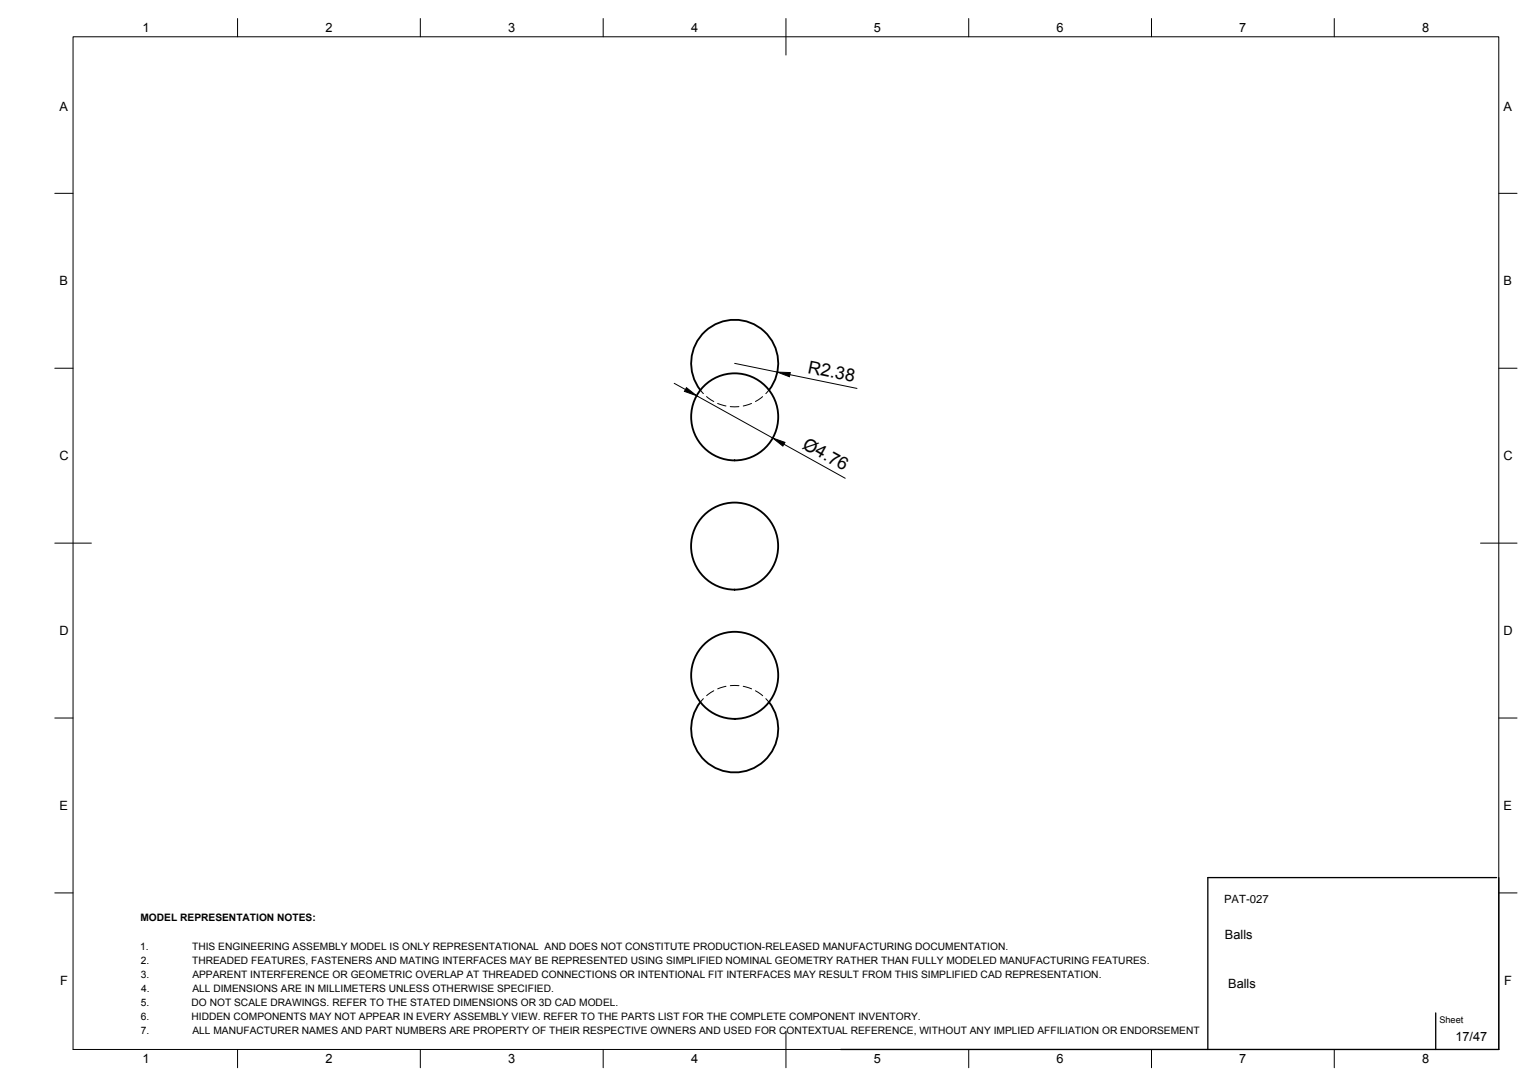
ISO-10303-21;
HEADER;
/* Generated by software containing ST-Developer
 * from STEP Tools, Inc. (www.steptools.com) 
 */

FILE_DESCRIPTION(
/* description */ ('Crank-driven oscillating fan base (mechanism only)'),

/* implementation_level */ '2;1');

FILE_NAME(
/* name */ 'Balls.step',
/* time_stamp */ '2026-10-28T03:25:00-07:00',
/* author */ (''),
/* organization */ (''),
/* preprocessor_version */ 'ST-DEVELOPER v20.2',
/* originating_system */ 'Autodesk Translation Framework v15.17.0.0',
/* authorisation */ '');

FILE_SCHEMA (('AUTOMOTIVE_DESIGN { 1 0 10303 214 3 1 1 }'));
ENDSEC;

DATA;
#10=MECHANICAL_DESIGN_GEOMETRIC_PRESENTATION_REPRESENTATION('',(#448,#449,#450,#451,#452,#453,#454,#455),#11916);
#275=SPHERICAL_SURFACE('',#6871,0.23815);
#276=SPHERICAL_SURFACE('',#6873,0.23815);
#277=SPHERICAL_SURFACE('',#6875,0.23815);
#278=SPHERICAL_SURFACE('',#6877,0.23815);
#279=SPHERICAL_SURFACE('',#6879,0.23815);
#280=SPHERICAL_SURFACE('',#6881,0.23815);
#281=SPHERICAL_SURFACE('',#6883,0.23815);
#282=SPHERICAL_SURFACE('',#6885,0.23815);
#368=SHAPE_REPRESENTATION_RELATIONSHIP('SRR','None',#12093,#408);
#408=ADVANCED_BREP_SHAPE_REPRESENTATION('',(#495,#496,#497,#498,#499,#500,
#501,#502),#11884);
#448=STYLED_ITEM('',(#12375),#495);
#449=STYLED_ITEM('',(#12375),#496);
#450=STYLED_ITEM('',(#12375),#497);
#451=STYLED_ITEM('',(#12375),#498);
#452=STYLED_ITEM('',(#12375),#499);
#453=STYLED_ITEM('',(#12375),#500);
#454=STYLED_ITEM('',(#12375),#501);
#455=STYLED_ITEM('',(#12375),#502);
#495=MANIFOLD_SOLID_BREP('Body1',#6079);
#496=MANIFOLD_SOLID_BREP('Body2',#6080);
#497=MANIFOLD_SOLID_BREP('Body3',#6081);
#498=MANIFOLD_SOLID_BREP('Body4',#6082);
#499=MANIFOLD_SOLID_BREP('Body5',#6083);
#500=MANIFOLD_SOLID_BREP('Body6',#6084);
#501=MANIFOLD_SOLID_BREP('Body7',#6085);
#502=MANIFOLD_SOLID_BREP('Body8',#6086);
#1026=FACE_OUTER_BOUND('',#1482,.T.);
#1027=FACE_OUTER_BOUND('',#1483,.T.);
#1028=FACE_OUTER_BOUND('',#1484,.T.);
#1029=FACE_OUTER_BOUND('',#1485,.T.);
#1030=FACE_OUTER_BOUND('',#1486,.T.);
#1031=FACE_OUTER_BOUND('',#1487,.T.);
#1032=FACE_OUTER_BOUND('',#1488,.T.);
#1033=FACE_OUTER_BOUND('',#1489,.T.);
#1482=EDGE_LOOP('',(#4668,#4669));
#1483=EDGE_LOOP('',(#4670,#4671));
#1484=EDGE_LOOP('',(#4672,#4673));
#1485=EDGE_LOOP('',(#4674,#4675));
#1486=EDGE_LOOP('',(#4676,#4677));
#1487=EDGE_LOOP('',(#4678,#4679));
#1488=EDGE_LOOP('',(#4680,#4681));
#1489=EDGE_LOOP('',(#4682,#4683));
#2621=CIRCLE('',#6872,0.23815);
#2622=CIRCLE('',#6874,0.23815);
#2623=CIRCLE('',#6876,0.23815);
#2624=CIRCLE('',#6878,0.23815);
#2625=CIRCLE('',#6880,0.23815);
#2626=CIRCLE('',#6882,0.23815);
#2627=CIRCLE('',#6884,0.23815);
#2628=CIRCLE('',#6886,0.23815);
#3028=VERTEX_POINT('',#10239);
#3029=VERTEX_POINT('',#10240);
#3030=VERTEX_POINT('',#10243);
#3031=VERTEX_POINT('',#10244);
#3032=VERTEX_POINT('',#10247);
#3033=VERTEX_POINT('',#10248);
#3034=VERTEX_POINT('',#10251);
#3035=VERTEX_POINT('',#10252);
#3036=VERTEX_POINT('',#10255);
#3037=VERTEX_POINT('',#10256);
#3038=VERTEX_POINT('',#10259);
#3039=VERTEX_POINT('',#10260);
#3040=VERTEX_POINT('',#10263);
#3041=VERTEX_POINT('',#10264);
#3042=VERTEX_POINT('',#10267);
#3043=VERTEX_POINT('',#10268);
#3629=EDGE_CURVE('',#3028,#3029,#2621,.T.);
#3630=EDGE_CURVE('',#3030,#3031,#2622,.T.);
#3631=EDGE_CURVE('',#3032,#3033,#2623,.T.);
#3632=EDGE_CURVE('',#3034,#3035,#2624,.T.);
#3633=EDGE_CURVE('',#3036,#3037,#2625,.T.);
#3634=EDGE_CURVE('',#3038,#3039,#2626,.T.);
#3635=EDGE_CURVE('',#3040,#3041,#2627,.T.);
#3636=EDGE_CURVE('',#3042,#3043,#2628,.T.);
#4668=ORIENTED_EDGE('',*,*,#3629,.T.);
#4669=ORIENTED_EDGE('',*,*,#3629,.F.);
#4670=ORIENTED_EDGE('',*,*,#3630,.T.);
#4671=ORIENTED_EDGE('',*,*,#3630,.F.);
#4672=ORIENTED_EDGE('',*,*,#3631,.T.);
#4673=ORIENTED_EDGE('',*,*,#3631,.F.);
#4674=ORIENTED_EDGE('',*,*,#3632,.T.);
#4675=ORIENTED_EDGE('',*,*,#3632,.F.);
#4676=ORIENTED_EDGE('',*,*,#3633,.T.);
#4677=ORIENTED_EDGE('',*,*,#3633,.F.);
#4678=ORIENTED_EDGE('',*,*,#3634,.T.);
#4679=ORIENTED_EDGE('',*,*,#3634,.F.);
#4680=ORIENTED_EDGE('',*,*,#3635,.T.);
#4681=ORIENTED_EDGE('',*,*,#3635,.F.);
#4682=ORIENTED_EDGE('',*,*,#3636,.T.);
#4683=ORIENTED_EDGE('',*,*,#3636,.F.);
#5832=ADVANCED_FACE('',(#1026),#275,.T.);
#5833=ADVANCED_FACE('',(#1027),#276,.T.);
#5834=ADVANCED_FACE('',(#1028),#277,.T.);
#5835=ADVANCED_FACE('',(#1029),#278,.T.);
#5836=ADVANCED_FACE('',(#1030),#279,.T.);
#5837=ADVANCED_FACE('',(#1031),#280,.T.);
#5838=ADVANCED_FACE('',(#1032),#281,.T.);
#5839=ADVANCED_FACE('',(#1033),#282,.T.);
#6079=CLOSED_SHELL('',(#5832));
#6080=CLOSED_SHELL('',(#5833));
#6081=CLOSED_SHELL('',(#5834));
#6082=CLOSED_SHELL('',(#5835));
#6083=CLOSED_SHELL('',(#5836));
#6084=CLOSED_SHELL('',(#5837));
#6085=CLOSED_SHELL('',(#5838));
#6086=CLOSED_SHELL('',(#5839));
#6870=AXIS2_PLACEMENT_3D('',#10237,#8168,#8169);
#6871=AXIS2_PLACEMENT_3D('',#10238,#8170,#8171);
#6872=AXIS2_PLACEMENT_3D('',#10241,#8172,#8173);
#6873=AXIS2_PLACEMENT_3D('',#10242,#8174,#8175);
#6874=AXIS2_PLACEMENT_3D('',#10245,#8176,#8177);
#6875=AXIS2_PLACEMENT_3D('',#10246,#8178,#8179);
#6876=AXIS2_PLACEMENT_3D('',#10249,#8180,#8181);
#6877=AXIS2_PLACEMENT_3D('',#10250,#8182,#8183);
#6878=AXIS2_PLACEMENT_3D('',#10253,#8184,#8185);
#6879=AXIS2_PLACEMENT_3D('',#10254,#8186,#8187);
#6880=AXIS2_PLACEMENT_3D('',#10257,#8188,#8189);
#6881=AXIS2_PLACEMENT_3D('',#10258,#8190,#8191);
#6882=AXIS2_PLACEMENT_3D('',#10261,#8192,#8193);
#6883=AXIS2_PLACEMENT_3D('',#10262,#8194,#8195);
#6884=AXIS2_PLACEMENT_3D('',#10265,#8196,#8197);
#6885=AXIS2_PLACEMENT_3D('',#10266,#8198,#8199);
#6886=AXIS2_PLACEMENT_3D('',#10269,#8200,#8201);
#8168=DIRECTION('axis',(0.,0.,1.));
#8169=DIRECTION('refdir',(1.,0.,0.));
#8170=DIRECTION('center_axis',(0.,0.,1.));
#8171=DIRECTION('ref_axis',(1.,0.,0.));
#8172=DIRECTION('center_axis',(1.22464679914735E-16,-1.,0.));
#8173=DIRECTION('ref_axis',(-1.,-1.22464679914735E-16,0.));
#8174=DIRECTION('center_axis',(0.707106781186548,0.,0.707106781186548));
#8175=DIRECTION('ref_axis',(0.707106781186548,0.,-0.707106781186548));
#8176=DIRECTION('center_axis',(8.65956056235494E-17,-1.,-8.65956056235493E-17));
#8177=DIRECTION('ref_axis',(-0.707106781186547,-1.22464679914735E-16,0.707106781186547));
#8178=DIRECTION('center_axis',(1.,0.,0.));
#8179=DIRECTION('ref_axis',(6.12323399573676E-17,0.,-1.));
#8180=DIRECTION('center_axis',(7.49879891330929E-33,-1.,-1.22464679914735E-16));
#8181=DIRECTION('ref_axis',(-6.12323399573676E-17,-1.22464679914735E-16,
1.));
#8182=DIRECTION('center_axis',(0.707106781186548,0.,-0.707106781186548));
#8183=DIRECTION('ref_axis',(-0.707106781186548,0.,-0.707106781186548));
#8184=DIRECTION('center_axis',(-8.65956056235493E-17,-1.,-8.65956056235494E-17));
#8185=DIRECTION('ref_axis',(0.707106781186547,-1.22464679914735E-16,0.707106781186547));
#8186=DIRECTION('center_axis',(0.,0.,-1.));
#8187=DIRECTION('ref_axis',(-1.,0.,-1.22464679914735E-16));
#8188=DIRECTION('center_axis',(-1.22464679914735E-16,-1.,-1.49975978266186E-32));
#8189=DIRECTION('ref_axis',(1.,-1.22464679914735E-16,1.22464679914735E-16));
#8190=DIRECTION('center_axis',(-0.707106781186547,0.,-0.707106781186548));
#8191=DIRECTION('ref_axis',(-0.707106781186548,0.,0.707106781186547));
#8192=DIRECTION('center_axis',(-8.65956056235493E-17,-1.,8.65956056235493E-17));
#8193=DIRECTION('ref_axis',(0.707106781186548,-1.22464679914735E-16,-0.707106781186547));
#8194=DIRECTION('center_axis',(-1.,0.,0.));
#8195=DIRECTION('ref_axis',(-1.83697019872103E-16,0.,1.));
#8196=DIRECTION('center_axis',(-2.24963967399279E-32,-1.,1.22464679914735E-16));
#8197=DIRECTION('ref_axis',(1.83697019872103E-16,-1.22464679914735E-16,
-1.));
#8198=DIRECTION('center_axis',(-0.707106781186548,0.,0.707106781186548));
#8199=DIRECTION('ref_axis',(0.707106781186547,0.,0.707106781186548));
#8200=DIRECTION('center_axis',(8.65956056235493E-17,-1.,8.65956056235493E-17));
#8201=DIRECTION('ref_axis',(-0.707106781186547,-1.22464679914735E-16,-0.707106781186548));
#10237=CARTESIAN_POINT('',(0.,0.,0.));
#10238=CARTESIAN_POINT('Origin',(1.,0.,0.));
#10239=CARTESIAN_POINT('',(1.,-1.78583896120461E-33,0.23815));
#10240=CARTESIAN_POINT('',(1.,-1.78583896120461E-33,-0.23815));
#10241=CARTESIAN_POINT('Origin',(1.,0.,0.));
#10242=CARTESIAN_POINT('Origin',(0.707106781186548,0.,-0.707106781186547));
#10243=CARTESIAN_POINT('',(0.875504261126124,-1.78583896120461E-33,-0.538709301246971));
#10244=CARTESIAN_POINT('',(0.538709301246971,-1.78583896120461E-33,-0.875504261126124));
#10245=CARTESIAN_POINT('Origin',(0.707106781186548,0.,-0.707106781186547));
#10246=CARTESIAN_POINT('Origin',(6.12323399573677E-17,0.,-1.));
#10247=CARTESIAN_POINT('',(0.23815,-1.78583896120461E-33,-1.));
#10248=CARTESIAN_POINT('',(-0.23815,-1.78583896120461E-33,-1.));
#10249=CARTESIAN_POINT('Origin',(6.12323399573677E-17,0.,-1.));
#10250=CARTESIAN_POINT('Origin',(-0.707106781186547,0.,-0.707106781186548));
#10251=CARTESIAN_POINT('',(-0.538709301246971,-1.78583896120461E-33,-0.875504261126124));
#10252=CARTESIAN_POINT('',(-0.875504261126124,-1.78583896120461E-33,-0.538709301246971));
#10253=CARTESIAN_POINT('Origin',(-0.707106781186547,0.,-0.707106781186548));
#10254=CARTESIAN_POINT('Origin',(-1.,0.,-1.22464679914735E-16));
#10255=CARTESIAN_POINT('',(-1.,-1.78583896120461E-33,-0.23815));
#10256=CARTESIAN_POINT('',(-1.,-1.78583896120461E-33,0.23815));
#10257=CARTESIAN_POINT('Origin',(-1.,0.,-1.22464679914735E-16));
#10258=CARTESIAN_POINT('Origin',(-0.707106781186548,0.,0.707106781186547));
#10259=CARTESIAN_POINT('',(-0.875504261126124,-7.94881478324376E-33,0.538709301246971));
#10260=CARTESIAN_POINT('',(-0.538709301246971,4.37713686083455E-33,0.875504261126124));
#10261=CARTESIAN_POINT('Origin',(-0.707106781186548,0.,0.707106781186547));
#10262=CARTESIAN_POINT('Origin',(-1.83697019872103E-16,0.,1.));
#10263=CARTESIAN_POINT('',(-0.23815,-1.78583896120461E-33,1.));
#10264=CARTESIAN_POINT('',(0.23815,-1.78583896120461E-33,1.));
#10265=CARTESIAN_POINT('Origin',(-1.83697019872103E-16,0.,1.));
#10266=CARTESIAN_POINT('Origin',(0.707106781186547,0.,0.707106781186548));
#10267=CARTESIAN_POINT('',(0.538709301246971,-4.86732687222419E-33,0.875504261126124));
#10268=CARTESIAN_POINT('',(0.875504261126124,1.29564894981497E-33,0.538709301246971));
#10269=CARTESIAN_POINT('Origin',(0.707106781186547,0.,0.707106781186548));
#11837=UNCERTAINTY_MEASURE_WITH_UNIT(LENGTH_MEASURE(0.001),#11917,
'DISTANCE_ACCURACY_VALUE',
'Maximum model space distance between geometric entities at asserted c
onnectivities');
#11869=UNCERTAINTY_MEASURE_WITH_UNIT(LENGTH_MEASURE(0.001),#11917,
'DISTANCE_ACCURACY_VALUE',
'Maximum model space distance between geometric entities at asserted c
onnectivities');
#11884=(
GEOMETRIC_REPRESENTATION_CONTEXT(3)
GLOBAL_UNCERTAINTY_ASSIGNED_CONTEXT((#11837))
GLOBAL_UNIT_ASSIGNED_CONTEXT((#11917,#11919,#11920))
REPRESENTATION_CONTEXT('','3D')
);
#11916=(
GEOMETRIC_REPRESENTATION_CONTEXT(3)
GLOBAL_UNCERTAINTY_ASSIGNED_CONTEXT((#11869))
GLOBAL_UNIT_ASSIGNED_CONTEXT((#11917,#11919,#11920))
REPRESENTATION_CONTEXT('','3D')
);
#11917=(
LENGTH_UNIT()
NAMED_UNIT(*)
SI_UNIT(.CENTI.,.METRE.)
);
#11919=(
NAMED_UNIT(*)
PLANE_ANGLE_UNIT()
SI_UNIT($,.RADIAN.)
);
#11920=(
NAMED_UNIT(*)
SI_UNIT($,.STERADIAN.)
SOLID_ANGLE_UNIT()
);
#11935=SHAPE_DEFINITION_REPRESENTATION(#11981,#12093);
#11981=PRODUCT_DEFINITION_SHAPE('',$,#12140);
#12093=SHAPE_REPRESENTATION('',(#6870),#11884);
#12125=PRODUCT_DEFINITION_CONTEXT('part definition',#12265,'design');
#12140=PRODUCT_DEFINITION('Balls','Balls',#12186,#12125);
#12186=PRODUCT_DEFINITION_FORMATION('',$,#12281);
#12265=APPLICATION_CONTEXT(
'Core Data for Automotive Mechanical Design Process');
#12266=PRODUCT_CONTEXT('part definition',#12265,'mechanical');
#12281=PRODUCT('Balls','Balls','Balls',(#12266));
#12369=COLOUR_RGB('Grey',0.48,0.52,0.57);
#12370=FILL_AREA_STYLE_COLOUR('',#12369);
#12371=FILL_AREA_STYLE('',(#12370));
#12372=SURFACE_STYLE_FILL_AREA(#12371);
#12373=SURFACE_SIDE_STYLE('',(#12372));
#12374=SURFACE_STYLE_USAGE(.BOTH.,#12373);
#12375=PRESENTATION_STYLE_ASSIGNMENT((#12374));
ENDSEC;
END-ISO-10303-21;
